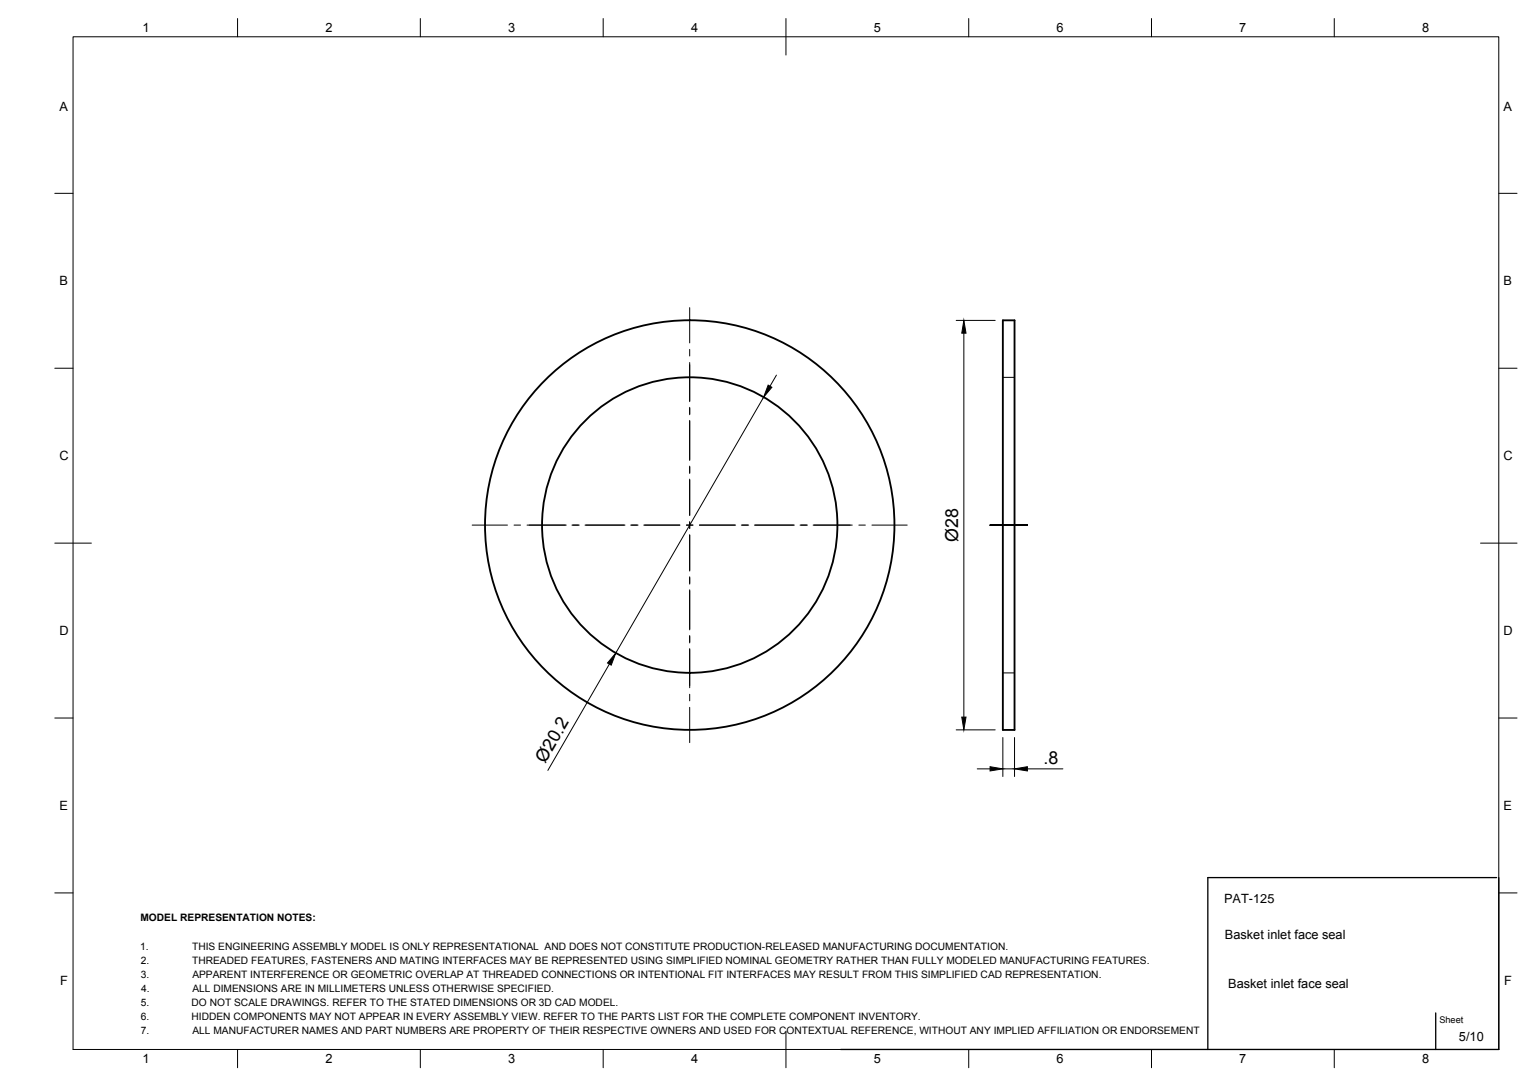
ISO-10303-21;
HEADER;
/* Generated by software containing ST-Developer
 * from STEP Tools, Inc. (www.steptools.com) 
 */

FILE_DESCRIPTION(
/* description */ ('Y-strainer with drain'),
/* implementation_level */ '2;1');

FILE_NAME(
/* name */ 'Basket inlet face seal.step',
/* time_stamp */ '2026-10-28T00:41:55-07:00',
/* author */ (''),
/* organization */ (''),
/* preprocessor_version */ 'ST-DEVELOPER v20.2',
/* originating_system */ 'Autodesk Translation Framework v15.17.0.0',
/* authorisation */ '');

FILE_SCHEMA (('AUTOMOTIVE_DESIGN { 1 0 10303 214 3 1 1 }'));
ENDSEC;

DATA;
#10=MECHANICAL_DESIGN_GEOMETRIC_PRESENTATION_REPRESENTATION('',(#95),#8864);
#77=SHAPE_REPRESENTATION_RELATIONSHIP('SRR','None',#8909,#86);
#86=ADVANCED_BREP_SHAPE_REPRESENTATION('',(#104),#8857);
#95=STYLED_ITEM('',(#9040),#104);
#104=MANIFOLD_SOLID_BREP('Body1',#3385);
#425=FACE_BOUND('',#865,.T.);
#426=FACE_BOUND('',#867,.T.);
#481=PLANE('',#3637);
#482=PLANE('',#3638);
#604=FACE_OUTER_BOUND('',#862,.T.);
#605=FACE_OUTER_BOUND('',#863,.T.);
#606=FACE_OUTER_BOUND('',#864,.T.);
#607=FACE_OUTER_BOUND('',#866,.T.);
#862=EDGE_LOOP('',(#2870,#2871,#2872,#2873));
#863=EDGE_LOOP('',(#2874,#2875,#2876,#2877));
#864=EDGE_LOOP('',(#2878));
#865=EDGE_LOOP('',(#2879));
#866=EDGE_LOOP('',(#2880));
#867=EDGE_LOOP('',(#2881));
#1041=LINE('',#8534,#1204);
#1042=LINE('',#8540,#1205);
#1204=VECTOR('',#4131,1.01);
#1205=VECTOR('',#4138,1.4);
#1327=CIRCLE('',#3632,1.01);
#1328=CIRCLE('',#3633,1.01);
#1329=CIRCLE('',#3635,1.4);
#1330=CIRCLE('',#3636,1.4);
#1633=VERTEX_POINT('',#8531);
#1634=VERTEX_POINT('',#8533);
#1635=VERTEX_POINT('',#8537);
#1636=VERTEX_POINT('',#8539);
#2059=EDGE_CURVE('',#1633,#1633,#1327,.T.);
#2060=EDGE_CURVE('',#1633,#1634,#1041,.T.);
#2061=EDGE_CURVE('',#1634,#1634,#1328,.T.);
#2062=EDGE_CURVE('',#1635,#1635,#1329,.T.);
#2063=EDGE_CURVE('',#1635,#1636,#1042,.T.);
#2064=EDGE_CURVE('',#1636,#1636,#1330,.T.);
#2870=ORIENTED_EDGE('',*,*,#2059,.F.);
#2871=ORIENTED_EDGE('',*,*,#2060,.T.);
#2872=ORIENTED_EDGE('',*,*,#2061,.T.);
#2873=ORIENTED_EDGE('',*,*,#2060,.F.);
#2874=ORIENTED_EDGE('',*,*,#2062,.F.);
#2875=ORIENTED_EDGE('',*,*,#2063,.T.);
#2876=ORIENTED_EDGE('',*,*,#2064,.T.);
#2877=ORIENTED_EDGE('',*,*,#2063,.F.);
#2878=ORIENTED_EDGE('',*,*,#2062,.T.);
#2879=ORIENTED_EDGE('',*,*,#2059,.T.);
#2880=ORIENTED_EDGE('',*,*,#2064,.F.);
#2881=ORIENTED_EDGE('',*,*,#2061,.F.);
#3208=CYLINDRICAL_SURFACE('',#3631,1.01);
#3209=CYLINDRICAL_SURFACE('',#3634,1.4);
#3315=ADVANCED_FACE('',(#604),#3208,.F.);
#3316=ADVANCED_FACE('',(#605),#3209,.T.);
#3317=ADVANCED_FACE('',(#606,#425),#481,.T.);
#3318=ADVANCED_FACE('',(#607,#426),#482,.F.);
#3385=CLOSED_SHELL('',(#3315,#3316,#3317,#3318));
#3630=AXIS2_PLACEMENT_3D('',#8529,#4125,#4126);
#3631=AXIS2_PLACEMENT_3D('',#8530,#4127,#4128);
#3632=AXIS2_PLACEMENT_3D('',#8532,#4129,#4130);
#3633=AXIS2_PLACEMENT_3D('',#8535,#4132,#4133);
#3634=AXIS2_PLACEMENT_3D('',#8536,#4134,#4135);
#3635=AXIS2_PLACEMENT_3D('',#8538,#4136,#4137);
#3636=AXIS2_PLACEMENT_3D('',#8541,#4139,#4140);
#3637=AXIS2_PLACEMENT_3D('',#8542,#4141,#4142);
#3638=AXIS2_PLACEMENT_3D('',#8543,#4143,#4144);
#4125=DIRECTION('axis',(0.,0.,1.));
#4126=DIRECTION('refdir',(1.,0.,0.));
#4127=DIRECTION('center_axis',(0.707106781186548,0.,-0.707106781186547));
#4128=DIRECTION('ref_axis',(-0.707106781186547,0.,-0.707106781186548));
#4129=DIRECTION('center_axis',(-0.707106781186548,0.,0.707106781186547));
#4130=DIRECTION('ref_axis',(-0.707106781186547,0.,-0.707106781186548));
#4131=DIRECTION('',(-0.707106781186548,0.,0.707106781186547));
#4132=DIRECTION('center_axis',(-0.707106781186548,0.,0.707106781186547));
#4133=DIRECTION('ref_axis',(-0.707106781186547,0.,-0.707106781186548));
#4134=DIRECTION('center_axis',(0.707106781186548,0.,-0.707106781186547));
#4135=DIRECTION('ref_axis',(-0.707106781186547,0.,-0.707106781186548));
#4136=DIRECTION('center_axis',(0.707106781186548,0.,-0.707106781186547));
#4137=DIRECTION('ref_axis',(-0.707106781186547,0.,-0.707106781186548));
#4138=DIRECTION('',(-0.707106781186548,0.,0.707106781186547));
#4139=DIRECTION('center_axis',(0.707106781186548,0.,-0.707106781186547));
#4140=DIRECTION('ref_axis',(-0.707106781186547,0.,-0.707106781186548));
#4141=DIRECTION('center_axis',(0.707106781186548,0.,-0.707106781186547));
#4142=DIRECTION('ref_axis',(-0.707106781186547,0.,-0.707106781186548));
#4143=DIRECTION('center_axis',(0.707106781186548,0.,-0.707106781186547));
#4144=DIRECTION('ref_axis',(-0.707106781186547,0.,-0.707106781186548));
#8529=CARTESIAN_POINT('',(0.,0.,0.));
#8530=CARTESIAN_POINT('Origin',(-0.575735931288071,0.,6.57573593128807));
#8531=CARTESIAN_POINT('',(0.195010460205266,-1.23689326713883E-16,7.23334523779156));
#8532=CARTESIAN_POINT('Origin',(-0.519167388793147,0.,6.51916738879315));
#8533=CARTESIAN_POINT('',(0.138441917710342,-1.23689326713883E-16,7.28991378028648));
#8534=CARTESIAN_POINT('',(0.138441917710342,-1.23689326713883E-16,7.28991378028648));
#8535=CARTESIAN_POINT('Origin',(-0.575735931288071,0.,6.57573593128807));
#8536=CARTESIAN_POINT('Origin',(-0.575735931288071,0.,6.57573593128807));
#8537=CARTESIAN_POINT('',(0.470782104868019,-1.71450551880629E-16,7.50911688245431));
#8538=CARTESIAN_POINT('Origin',(-0.519167388793147,0.,6.51916738879315));
#8539=CARTESIAN_POINT('',(0.414213562373095,-1.71450551880629E-16,7.56568542494924));
#8540=CARTESIAN_POINT('',(0.414213562373095,-1.71450551880629E-16,7.56568542494924));
#8541=CARTESIAN_POINT('Origin',(-0.575735931288071,0.,6.57573593128807));
#8542=CARTESIAN_POINT('Origin',(-0.519167388793147,0.,6.51916738879315));
#8543=CARTESIAN_POINT('Origin',(-0.575735931288071,0.,6.57573593128807));
#8845=UNCERTAINTY_MEASURE_WITH_UNIT(LENGTH_MEASURE(0.001),#8865,
'DISTANCE_ACCURACY_VALUE',
'Maximum model space distance between geometric entities at asserted c
onnectivities');
#8852=UNCERTAINTY_MEASURE_WITH_UNIT(LENGTH_MEASURE(0.001),#8865,
'DISTANCE_ACCURACY_VALUE',
'Maximum model space distance between geometric entities at asserted c
onnectivities');
#8857=(
GEOMETRIC_REPRESENTATION_CONTEXT(3)
GLOBAL_UNCERTAINTY_ASSIGNED_CONTEXT((#8845))
GLOBAL_UNIT_ASSIGNED_CONTEXT((#8865,#8867,#8868))
REPRESENTATION_CONTEXT('','3D')
);
#8864=(
GEOMETRIC_REPRESENTATION_CONTEXT(3)
GLOBAL_UNCERTAINTY_ASSIGNED_CONTEXT((#8852))
GLOBAL_UNIT_ASSIGNED_CONTEXT((#8865,#8867,#8868))
REPRESENTATION_CONTEXT('','3D')
);
#8865=(
LENGTH_UNIT()
NAMED_UNIT(*)
SI_UNIT(.CENTI.,.METRE.)
);
#8867=(
NAMED_UNIT(*)
PLANE_ANGLE_UNIT()
SI_UNIT($,.RADIAN.)
);
#8868=(
NAMED_UNIT(*)
SI_UNIT($,.STERADIAN.)
SOLID_ANGLE_UNIT()
);
#8873=SHAPE_DEFINITION_REPRESENTATION(#8884,#8909);
#8884=PRODUCT_DEFINITION_SHAPE('',$,#8921);
#8909=SHAPE_REPRESENTATION('',(#3630),#8857);
#8916=PRODUCT_DEFINITION_CONTEXT('part definition',#8951,'design');
#8921=PRODUCT_DEFINITION('Basket inlet face seal',
'Basket inlet face seal',#8932,#8916);
#8932=PRODUCT_DEFINITION_FORMATION('',$,#8957);
#8951=APPLICATION_CONTEXT(
'Core Data for Automotive Mechanical Design Process');
#8952=PRODUCT_CONTEXT('part definition',#8951,'mechanical');
#8957=PRODUCT('Basket inlet face seal','Basket inlet face seal',
'Basket inlet face seal',(#8952));
#9034=COLOUR_RGB('Black',0.12,0.14,0.17);
#9035=FILL_AREA_STYLE_COLOUR('',#9034);
#9036=FILL_AREA_STYLE('',(#9035));
#9037=SURFACE_STYLE_FILL_AREA(#9036);
#9038=SURFACE_SIDE_STYLE('',(#9037));
#9039=SURFACE_STYLE_USAGE(.BOTH.,#9038);
#9040=PRESENTATION_STYLE_ASSIGNMENT((#9039));
ENDSEC;
END-ISO-10303-21;
